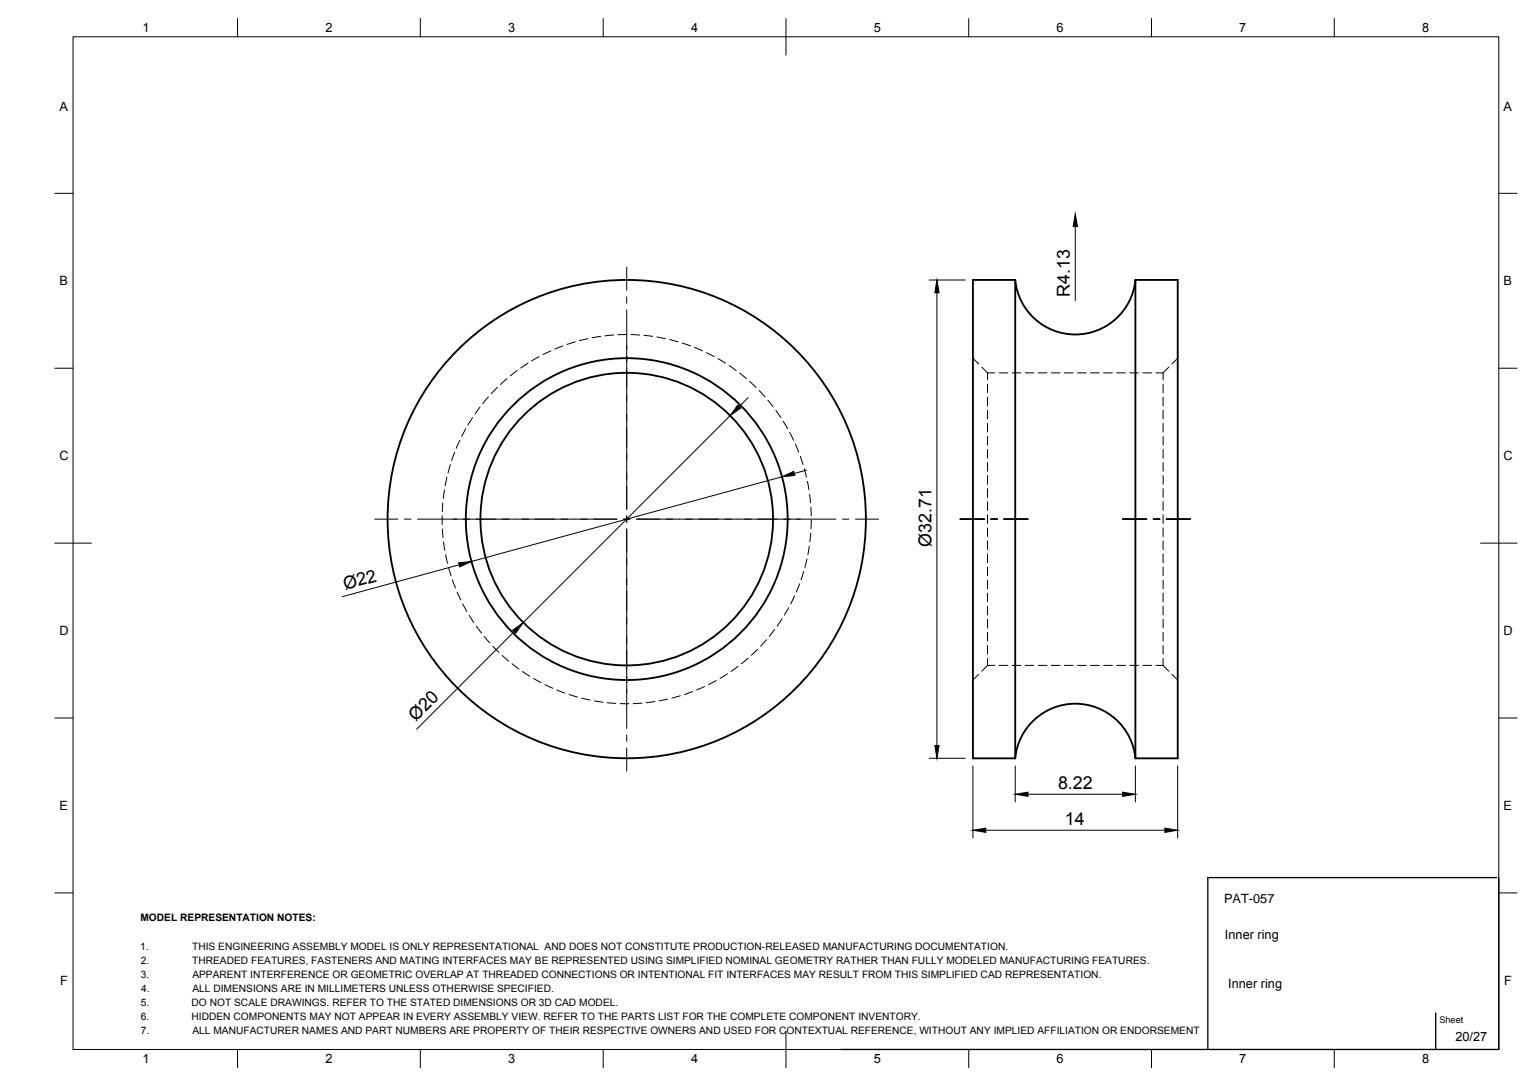
ISO-10303-21;
HEADER;
/* Generated by software containing ST-Developer
 * from STEP Tools, Inc. (www.steptools.com) 
 */

FILE_DESCRIPTION(
/* description */ ('Bearing-mounted hook block'),
/* implementation_level */ '2;1');

FILE_NAME(
/* name */ 'Inner ring.step',
/* time_stamp */ '2026-10-28T22:30:11-07:00',
/* author */ (''),
/* organization */ (''),
/* preprocessor_version */ 'ST-DEVELOPER v20.2',
/* originating_system */ 'Autodesk Translation Framework v15.17.0.0',
/* authorisation */ '');

FILE_SCHEMA (('AUTOMOTIVE_DESIGN { 1 0 10303 214 3 1 1 }'));
ENDSEC;

DATA;
#10=MECHANICAL_DESIGN_GEOMETRIC_PRESENTATION_REPRESENTATION('',(#337),#7609);
#45=TOROIDAL_SURFACE('',#4505,1.675,0.412776);
#262=CONICAL_SURFACE('',#4516,1.05,0.785398163397449);
#263=CONICAL_SURFACE('',#4523,1.05,0.785398163397449);
#289=SHAPE_REPRESENTATION_RELATIONSHIP('SRR','None',#7738,#313);
#313=ADVANCED_BREP_SHAPE_REPRESENTATION('',(#367),#7598);
#337=STYLED_ITEM('',(#7931),#367);
#367=MANIFOLD_SOLID_BREP('Body1',#3935);
#525=LINE('',#6712,#755);
#526=LINE('',#6718,#756);
#527=LINE('',#6722,#757);
#528=LINE('',#6728,#758);
#529=LINE('',#6733,#759);
#755=VECTOR('',#5484,1.63531);
#756=VECTOR('',#5491,1.);
#757=VECTOR('',#5496,1.05);
#758=VECTOR('',#5505,1.63531);
#759=VECTOR('',#5512,1.05);
#892=CYLINDRICAL_SURFACE('',#4511,1.63531);
#893=CYLINDRICAL_SURFACE('',#4513,1.);
#894=CYLINDRICAL_SURFACE('',#4519,1.63531);
#974=FACE_BOUND('',#1425,.T.);
#975=FACE_BOUND('',#1428,.T.);
#1131=FACE_OUTER_BOUND('',#1420,.T.);
#1132=FACE_OUTER_BOUND('',#1421,.T.);
#1133=FACE_OUTER_BOUND('',#1422,.T.);
#1134=FACE_OUTER_BOUND('',#1423,.T.);
#1135=FACE_OUTER_BOUND('',#1424,.T.);
#1136=FACE_OUTER_BOUND('',#1426,.T.);
#1137=FACE_OUTER_BOUND('',#1427,.T.);
#1138=FACE_OUTER_BOUND('',#1429,.T.);
#1420=EDGE_LOOP('',(#3124,#3125,#3126,#3127,#3128,#3129));
#1421=EDGE_LOOP('',(#3130,#3131,#3132,#3133,#3134));
#1422=EDGE_LOOP('',(#3135,#3136,#3137,#3138));
#1423=EDGE_LOOP('',(#3139,#3140,#3141,#3142));
#1424=EDGE_LOOP('',(#3143));
#1425=EDGE_LOOP('',(#3144));
#1426=EDGE_LOOP('',(#3145,#3146,#3147,#3148,#3149));
#1427=EDGE_LOOP('',(#3150));
#1428=EDGE_LOOP('',(#3151));
#1429=EDGE_LOOP('',(#3152,#3153,#3154,#3155));
#1667=CIRCLE('',#4506,1.63531);
#1668=CIRCLE('',#4507,1.63531);
#1669=CIRCLE('',#4508,0.412776);
#1670=CIRCLE('',#4509,1.63531);
#1671=CIRCLE('',#4510,1.63531);
#1672=CIRCLE('',#4512,1.63531);
#1673=CIRCLE('',#4514,1.);
#1674=CIRCLE('',#4515,1.);
#1675=CIRCLE('',#4517,1.1);
#1676=CIRCLE('',#4520,1.63531);
#1677=CIRCLE('',#4522,1.1);
#1952=VERTEX_POINT('',#6701);
#1953=VERTEX_POINT('',#6702);
#1954=VERTEX_POINT('',#6705);
#1955=VERTEX_POINT('',#6707);
#1956=VERTEX_POINT('',#6711);
#1957=VERTEX_POINT('',#6715);
#1958=VERTEX_POINT('',#6717);
#1959=VERTEX_POINT('',#6721);
#1960=VERTEX_POINT('',#6726);
#1961=VERTEX_POINT('',#6730);
#2372=EDGE_CURVE('',#1952,#1953,#1667,.T.);
#2373=EDGE_CURVE('',#1953,#1952,#1668,.T.);
#2374=EDGE_CURVE('',#1953,#1954,#1669,.T.);
#2375=EDGE_CURVE('',#1955,#1954,#1670,.T.);
#2376=EDGE_CURVE('',#1954,#1955,#1671,.T.);
#2377=EDGE_CURVE('',#1955,#1956,#525,.T.);
#2378=EDGE_CURVE('',#1956,#1956,#1672,.T.);
#2379=EDGE_CURVE('',#1957,#1957,#1673,.T.);
#2380=EDGE_CURVE('',#1957,#1958,#526,.T.);
#2381=EDGE_CURVE('',#1958,#1958,#1674,.T.);
#2382=EDGE_CURVE('',#1958,#1959,#527,.T.);
#2383=EDGE_CURVE('',#1959,#1959,#1675,.T.);
#2384=EDGE_CURVE('',#1960,#1960,#1676,.T.);
#2385=EDGE_CURVE('',#1960,#1952,#528,.T.);
#2386=EDGE_CURVE('',#1961,#1961,#1677,.T.);
#2387=EDGE_CURVE('',#1961,#1957,#529,.T.);
#3124=ORIENTED_EDGE('',*,*,#2372,.F.);
#3125=ORIENTED_EDGE('',*,*,#2373,.F.);
#3126=ORIENTED_EDGE('',*,*,#2374,.T.);
#3127=ORIENTED_EDGE('',*,*,#2375,.F.);
#3128=ORIENTED_EDGE('',*,*,#2376,.F.);
#3129=ORIENTED_EDGE('',*,*,#2374,.F.);
#3130=ORIENTED_EDGE('',*,*,#2375,.T.);
#3131=ORIENTED_EDGE('',*,*,#2376,.T.);
#3132=ORIENTED_EDGE('',*,*,#2377,.T.);
#3133=ORIENTED_EDGE('',*,*,#2378,.T.);
#3134=ORIENTED_EDGE('',*,*,#2377,.F.);
#3135=ORIENTED_EDGE('',*,*,#2379,.T.);
#3136=ORIENTED_EDGE('',*,*,#2380,.T.);
#3137=ORIENTED_EDGE('',*,*,#2381,.F.);
#3138=ORIENTED_EDGE('',*,*,#2380,.F.);
#3139=ORIENTED_EDGE('',*,*,#2381,.T.);
#3140=ORIENTED_EDGE('',*,*,#2382,.T.);
#3141=ORIENTED_EDGE('',*,*,#2383,.F.);
#3142=ORIENTED_EDGE('',*,*,#2382,.F.);
#3143=ORIENTED_EDGE('',*,*,#2378,.F.);
#3144=ORIENTED_EDGE('',*,*,#2383,.T.);
#3145=ORIENTED_EDGE('',*,*,#2384,.F.);
#3146=ORIENTED_EDGE('',*,*,#2385,.T.);
#3147=ORIENTED_EDGE('',*,*,#2372,.T.);
#3148=ORIENTED_EDGE('',*,*,#2373,.T.);
#3149=ORIENTED_EDGE('',*,*,#2385,.F.);
#3150=ORIENTED_EDGE('',*,*,#2384,.T.);
#3151=ORIENTED_EDGE('',*,*,#2386,.F.);
#3152=ORIENTED_EDGE('',*,*,#2386,.T.);
#3153=ORIENTED_EDGE('',*,*,#2387,.T.);
#3154=ORIENTED_EDGE('',*,*,#2379,.F.);
#3155=ORIENTED_EDGE('',*,*,#2387,.F.);
#3631=PLANE('',#4518);
#3632=PLANE('',#4521);
#3813=ADVANCED_FACE('',(#1131),#45,.F.);
#3814=ADVANCED_FACE('',(#1132),#892,.T.);
#3815=ADVANCED_FACE('',(#1133),#893,.F.);
#3816=ADVANCED_FACE('',(#1134),#262,.F.);
#3817=ADVANCED_FACE('',(#1135,#974),#3631,.T.);
#3818=ADVANCED_FACE('',(#1136),#894,.T.);
#3819=ADVANCED_FACE('',(#1137,#975),#3632,.T.);
#3820=ADVANCED_FACE('',(#1138),#263,.F.);
#3935=CLOSED_SHELL('',(#3813,#3814,#3815,#3816,#3817,#3818,#3819,#3820));
#4504=AXIS2_PLACEMENT_3D('',#6699,#5468,#5469);
#4505=AXIS2_PLACEMENT_3D('',#6700,#5470,#5471);
#4506=AXIS2_PLACEMENT_3D('',#6703,#5472,#5473);
#4507=AXIS2_PLACEMENT_3D('',#6704,#5474,#5475);
#4508=AXIS2_PLACEMENT_3D('',#6706,#5476,#5477);
#4509=AXIS2_PLACEMENT_3D('',#6708,#5478,#5479);
#4510=AXIS2_PLACEMENT_3D('',#6709,#5480,#5481);
#4511=AXIS2_PLACEMENT_3D('',#6710,#5482,#5483);
#4512=AXIS2_PLACEMENT_3D('',#6713,#5485,#5486);
#4513=AXIS2_PLACEMENT_3D('',#6714,#5487,#5488);
#4514=AXIS2_PLACEMENT_3D('',#6716,#5489,#5490);
#4515=AXIS2_PLACEMENT_3D('',#6719,#5492,#5493);
#4516=AXIS2_PLACEMENT_3D('',#6720,#5494,#5495);
#4517=AXIS2_PLACEMENT_3D('',#6723,#5497,#5498);
#4518=AXIS2_PLACEMENT_3D('',#6724,#5499,#5500);
#4519=AXIS2_PLACEMENT_3D('',#6725,#5501,#5502);
#4520=AXIS2_PLACEMENT_3D('',#6727,#5503,#5504);
#4521=AXIS2_PLACEMENT_3D('',#6729,#5506,#5507);
#4522=AXIS2_PLACEMENT_3D('',#6731,#5508,#5509);
#4523=AXIS2_PLACEMENT_3D('',#6732,#5510,#5511);
#5468=DIRECTION('axis',(0.,0.,1.));
#5469=DIRECTION('refdir',(1.,0.,0.));
#5470=DIRECTION('center_axis',(0.,-1.,0.));
#5471=DIRECTION('ref_axis',(0.,0.,-1.));
#5472=DIRECTION('center_axis',(0.,-1.,0.));
#5473=DIRECTION('ref_axis',(1.,0.,0.));
#5474=DIRECTION('center_axis',(0.,-1.,0.));
#5475=DIRECTION('ref_axis',(1.,0.,0.));
#5476=DIRECTION('center_axis',(1.,0.,1.22464679914735E-16));
#5477=DIRECTION('ref_axis',(-1.22464679914735E-16,0.,1.));
#5478=DIRECTION('center_axis',(0.,1.,0.));
#5479=DIRECTION('ref_axis',(1.,0.,0.));
#5480=DIRECTION('center_axis',(0.,1.,0.));
#5481=DIRECTION('ref_axis',(1.,0.,0.));
#5482=DIRECTION('center_axis',(0.,-1.,0.));
#5483=DIRECTION('ref_axis',(1.,0.,0.));
#5484=DIRECTION('',(0.,1.,0.));
#5485=DIRECTION('center_axis',(0.,-1.,0.));
#5486=DIRECTION('ref_axis',(1.,0.,0.));
#5487=DIRECTION('center_axis',(0.,-1.,0.));
#5488=DIRECTION('ref_axis',(1.,0.,0.));
#5489=DIRECTION('center_axis',(0.,-1.,0.));
#5490=DIRECTION('ref_axis',(1.,0.,0.));
#5491=DIRECTION('',(0.,1.,0.));
#5492=DIRECTION('center_axis',(0.,-1.,0.));
#5493=DIRECTION('ref_axis',(1.,0.,0.));
#5494=DIRECTION('center_axis',(0.,1.,0.));
#5495=DIRECTION('ref_axis',(1.,0.,0.));
#5496=DIRECTION('',(-0.707106781186548,0.707106781186547,-8.65956056235494E-17));
#5497=DIRECTION('center_axis',(0.,-1.,0.));
#5498=DIRECTION('ref_axis',(1.,0.,0.));
#5499=DIRECTION('center_axis',(0.,1.,0.));
#5500=DIRECTION('ref_axis',(0.,0.,1.));
#5501=DIRECTION('center_axis',(0.,-1.,0.));
#5502=DIRECTION('ref_axis',(1.,0.,0.));
#5503=DIRECTION('center_axis',(0.,-1.,0.));
#5504=DIRECTION('ref_axis',(1.,0.,0.));
#5505=DIRECTION('',(0.,1.,0.));
#5506=DIRECTION('center_axis',(0.,-1.,0.));
#5507=DIRECTION('ref_axis',(0.,0.,-1.));
#5508=DIRECTION('center_axis',(0.,-1.,0.));
#5509=DIRECTION('ref_axis',(1.,0.,0.));
#5510=DIRECTION('center_axis',(0.,-1.,0.));
#5511=DIRECTION('ref_axis',(1.,0.,0.));
#5512=DIRECTION('',(0.707106781186548,0.707106781186547,8.65956056235494E-17));
#6699=CARTESIAN_POINT('',(0.,0.,0.));
#6700=CARTESIAN_POINT('Origin',(0.,0.,0.));
#6701=CARTESIAN_POINT('',(-1.63531,-0.410863395882378,-2.00267715711366E-16));
#6702=CARTESIAN_POINT('',(-2.00267715711366E-16,-0.410863395882378,1.63531));
#6703=CARTESIAN_POINT('Origin',(0.,-0.410863395882378,0.));
#6704=CARTESIAN_POINT('Origin',(0.,-0.410863395882378,0.));
#6705=CARTESIAN_POINT('',(-2.00267715711366E-16,0.410863395882378,1.63531));
#6706=CARTESIAN_POINT('Origin',(-2.05128338857182E-16,0.,1.675));
#6707=CARTESIAN_POINT('',(-1.63531,0.410863395882378,2.00267715711366E-16));
#6708=CARTESIAN_POINT('Origin',(0.,0.410863395882378,0.));
#6709=CARTESIAN_POINT('Origin',(0.,0.410863395882378,0.));
#6710=CARTESIAN_POINT('Origin',(0.,0.,0.));
#6711=CARTESIAN_POINT('',(-1.63531,0.7,-2.00267715711366E-16));
#6712=CARTESIAN_POINT('',(-1.63531,0.,-2.00267715711366E-16));
#6713=CARTESIAN_POINT('Origin',(0.,0.7,0.));
#6714=CARTESIAN_POINT('Origin',(0.,0.,0.));
#6715=CARTESIAN_POINT('',(-1.,-0.6,-1.22464679914735E-16));
#6716=CARTESIAN_POINT('Origin',(0.,-0.6,0.));
#6717=CARTESIAN_POINT('',(-1.,0.6,-1.22464679914735E-16));
#6718=CARTESIAN_POINT('',(-1.,0.,-1.22464679914735E-16));
#6719=CARTESIAN_POINT('Origin',(0.,0.6,0.));
#6720=CARTESIAN_POINT('Origin',(0.,0.65,0.));
#6721=CARTESIAN_POINT('',(-1.1,0.7,-1.34711147906209E-16));
#6722=CARTESIAN_POINT('',(-1.05,0.65,-1.28587913910472E-16));
#6723=CARTESIAN_POINT('Origin',(0.,0.7,0.));
#6724=CARTESIAN_POINT('Origin',(1.63531,0.7,0.));
#6725=CARTESIAN_POINT('Origin',(0.,0.,0.));
#6726=CARTESIAN_POINT('',(-1.63531,-0.7,-2.00267715711366E-16));
#6727=CARTESIAN_POINT('Origin',(0.,-0.7,0.));
#6728=CARTESIAN_POINT('',(-1.63531,0.,-2.00267715711366E-16));
#6729=CARTESIAN_POINT('Origin',(1.1,-0.7,0.));
#6730=CARTESIAN_POINT('',(-1.1,-0.7,-1.34711147906209E-16));
#6731=CARTESIAN_POINT('Origin',(0.,-0.7,0.));
#6732=CARTESIAN_POINT('Origin',(0.,-0.65,0.));
#6733=CARTESIAN_POINT('',(-1.05,-0.65,-1.28587913910472E-16));
#7568=UNCERTAINTY_MEASURE_WITH_UNIT(LENGTH_MEASURE(0.001),#7610,
'DISTANCE_ACCURACY_VALUE',
'Maximum model space distance between geometric entities at asserted c
onnectivities');
#7579=UNCERTAINTY_MEASURE_WITH_UNIT(LENGTH_MEASURE(0.001),#7610,
'DISTANCE_ACCURACY_VALUE',
'Maximum model space distance between geometric entities at asserted c
onnectivities');
#7598=(
GEOMETRIC_REPRESENTATION_CONTEXT(3)
GLOBAL_UNCERTAINTY_ASSIGNED_CONTEXT((#7568))
GLOBAL_UNIT_ASSIGNED_CONTEXT((#7610,#7612,#7613))
REPRESENTATION_CONTEXT('','3D')
);
#7609=(
GEOMETRIC_REPRESENTATION_CONTEXT(3)
GLOBAL_UNCERTAINTY_ASSIGNED_CONTEXT((#7579))
GLOBAL_UNIT_ASSIGNED_CONTEXT((#7610,#7612,#7613))
REPRESENTATION_CONTEXT('','3D')
);
#7610=(
LENGTH_UNIT()
NAMED_UNIT(*)
SI_UNIT(.CENTI.,.METRE.)
);
#7612=(
NAMED_UNIT(*)
PLANE_ANGLE_UNIT()
SI_UNIT($,.RADIAN.)
);
#7613=(
NAMED_UNIT(*)
SI_UNIT($,.STERADIAN.)
SOLID_ANGLE_UNIT()
);
#7632=SHAPE_DEFINITION_REPRESENTATION(#7684,#7738);
#7684=PRODUCT_DEFINITION_SHAPE('',$,#7768);
#7738=SHAPE_REPRESENTATION('',(#4504),#7598);
#7749=PRODUCT_DEFINITION_CONTEXT('part definition',#7838,'design');
#7768=PRODUCT_DEFINITION('Inner ring','Inner ring',#7797,#7749);
#7797=PRODUCT_DEFINITION_FORMATION('',$,#7858);
#7838=APPLICATION_CONTEXT(
'Core Data for Automotive Mechanical Design Process');
#7839=PRODUCT_CONTEXT('part definition',#7838,'mechanical');
#7858=PRODUCT('Inner ring','Inner ring','Inner ring',(#7839));
#7925=COLOUR_RGB('Grey',0.48,0.52,0.57);
#7926=FILL_AREA_STYLE_COLOUR('',#7925);
#7927=FILL_AREA_STYLE('',(#7926));
#7928=SURFACE_STYLE_FILL_AREA(#7927);
#7929=SURFACE_SIDE_STYLE('',(#7928));
#7930=SURFACE_STYLE_USAGE(.BOTH.,#7929);
#7931=PRESENTATION_STYLE_ASSIGNMENT((#7930));
ENDSEC;
END-ISO-10303-21;
